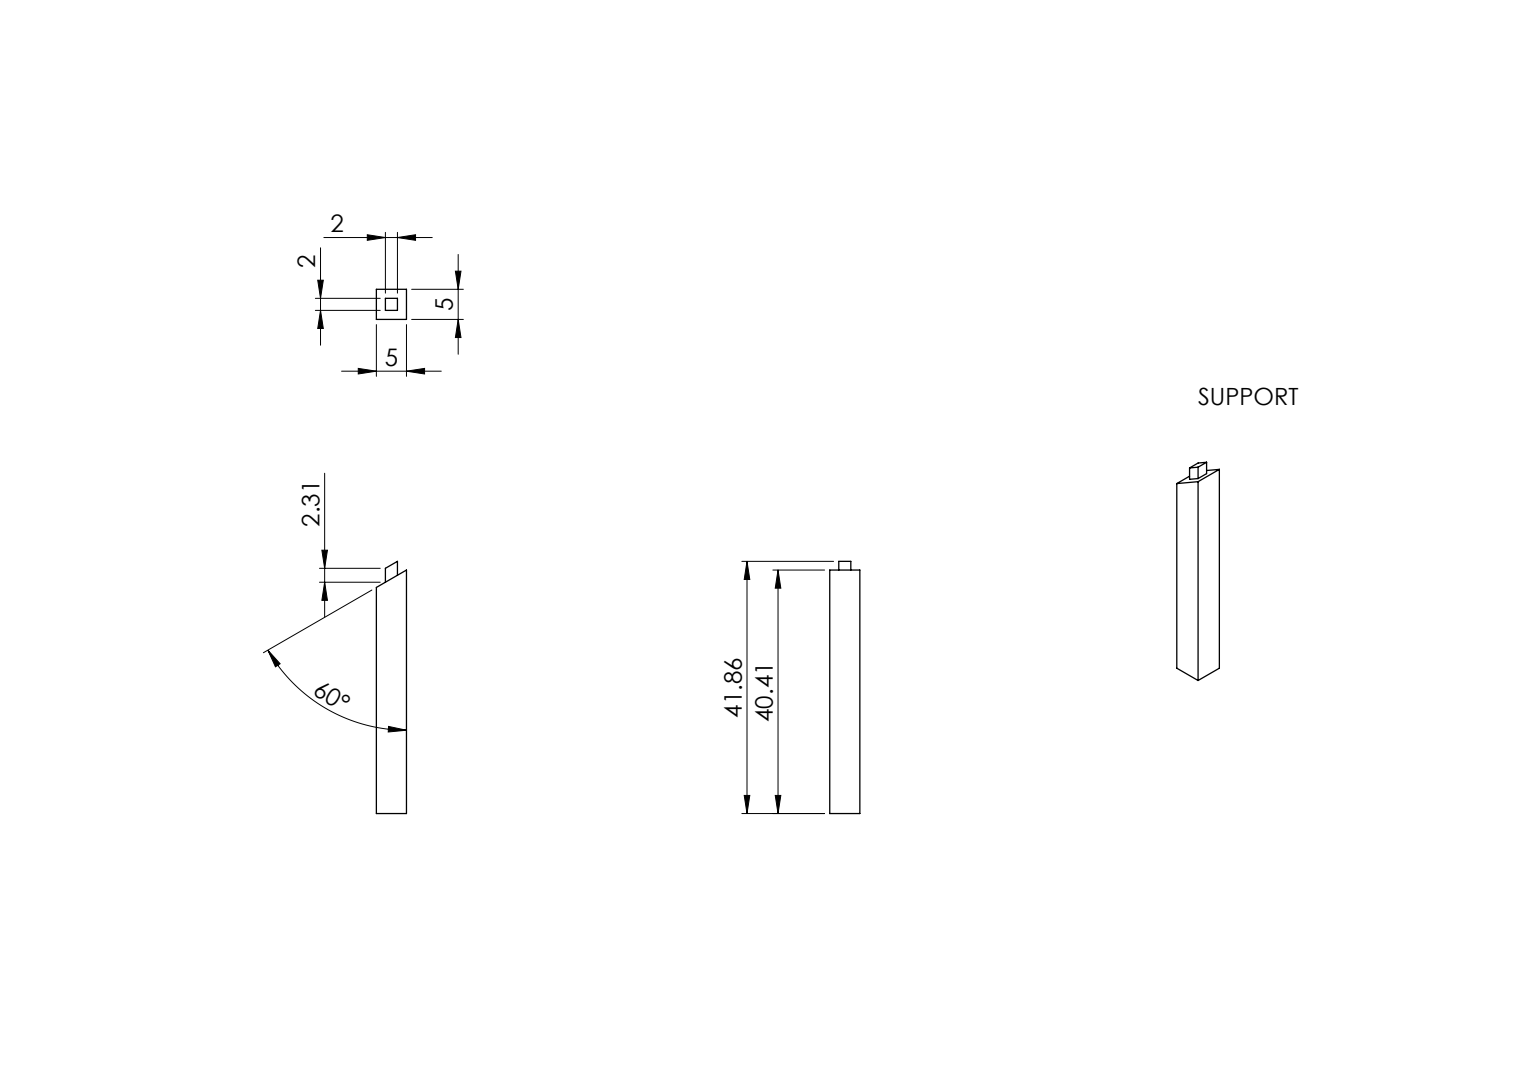
ISO-10303-21;
HEADER;
FILE_DESCRIPTION (('STEP AP214'),
    '1' );
FILE_NAME ('support.step',
    '2026-10-26T05:17:54',
    ( '' ),
    ( '' ),
    'SwSTEP 2.0',
    'SolidWorks 2026',
    '' );
FILE_SCHEMA (( 'AUTOMOTIVE_DESIGN' ));
ENDSEC;

DATA;
#17=CARTESIAN_POINT ( 'NONE',  ( 7.500000000000000000, 34.99999999999999289, -1.499999999999999556 ) ) ;
#43=ORIENTED_EDGE ( 'NONE', *, *, #1360, .T. ) ;
#55=APPLICATION_CONTEXT ( 'automotive_design' ) ;
#65=ORIENTED_EDGE ( 'NONE', *, *, #9345, .T. ) ;
#128=DIRECTION ( 'NONE',  ( 0.000000000000000000, 0.000000000000000000, -1.000000000000000000 ) ) ;
#162=ORIENTED_EDGE ( 'NONE', *, *, #11234, .F. ) ;
#197=DIRECTION ( 'NONE',  ( -0.000000000000000000, -1.000000000000000000, -0.000000000000000000 ) ) ;
#254=EDGE_CURVE ( 'NONE', #5137, #10011, #5741, .T. ) ;
#287=ADVANCED_FACE ( 'NONE', ( #7172 ), #1536, .F. ) ;
#303=DIRECTION ( 'NONE',  ( -1.000000000000000000, 0.000000000000000000, 4.336808689942017243E-16 ) ) ;
#312=ORIENTED_EDGE ( 'NONE', *, *, #4163, .F. ) ;
#338=ADVANCED_FACE ( 'NONE', ( #7108, #5337 ), #2214, .T. ) ;
#342=VECTOR ( 'NONE', #6084, 1000.000000000000000 ) ;
#366=LINE ( 'NONE', #8567, #6016 ) ;
#411=DIRECTION ( 'NONE',  ( -0.000000000000000000, 1.000000000000000000, -0.000000000000000000 ) ) ;
#459=DIRECTION ( 'NONE',  ( 0.000000000000000000, 0.000000000000000000, -1.000000000000000000 ) ) ;
#466=( GEOMETRIC_REPRESENTATION_CONTEXT ( 3 ) GLOBAL_UNCERTAINTY_ASSIGNED_CONTEXT ( ( #584 ) ) GLOBAL_UNIT_ASSIGNED_CONTEXT ( ( #1408, #547, #9650 ) ) REPRESENTATION_CONTEXT ( 'NONE', 'WORKASPACE' ) );
#522=DIRECTION ( 'NONE',  ( -0.000000000000000000, -1.000000000000000000, -0.000000000000000000 ) ) ;
#547=( NAMED_UNIT ( * ) PLANE_ANGLE_UNIT ( ) SI_UNIT ( $, .RADIAN. ) );
#559=DIRECTION ( 'NONE',  ( 1.000000000000000000, -0.000000000000000000, 0.000000000000000000 ) ) ;
#563=ORIENTED_EDGE ( 'NONE', *, *, #5905, .F. ) ;
#584=UNCERTAINTY_MEASURE_WITH_UNIT (LENGTH_MEASURE( 1.000000000000000082E-05 ), #1408, 'distance_accuracy_value', 'NONE');
#592=ORIENTED_EDGE ( 'NONE', *, *, #5905, .T. ) ;
#593=ADVANCED_FACE ( 'NONE', ( #5912, #5791 ), #3774, .T. ) ;
#615=( NAMED_UNIT ( * ) SI_UNIT ( $, .STERADIAN. ) SOLID_ANGLE_UNIT ( ) );
#628=LINE ( 'NONE', #4760, #11001 ) ;
#659=CARTESIAN_POINT ( 'NONE',  ( 6.499999999999999112, 68.39379290111055809, 2.999999999999960032 ) ) ;
#674=DIRECTION ( 'NONE',  ( -0.000000000000000000, 1.000000000000000000, -0.000000000000000000 ) ) ;
#682=CARTESIAN_POINT ( 'NONE',  ( 7.500000000000000000, 30.00000000000000000, 0.000000000000000000 ) ) ;
#692=LINE ( 'NONE', #4702, #11877 ) ;
#733=CARTESIAN_POINT ( 'NONE',  ( -61.00000000000000711, 26.13129029178200469, 0.9999999999999926725 ) ) ;
#790=DIRECTION ( 'NONE',  ( -1.084202172485503571E-16, 0.000000000000000000, 1.000000000000000000 ) ) ;
#872=CYLINDRICAL_SURFACE ( 'NONE', #11788, 1.499999999999999556 ) ;
#904=APPLICATION_CONTEXT ( 'automotive_design' ) ;
#954=ADVANCED_FACE ( 'NONE', ( #9768 ), #6949, .T. ) ;
#969=ORIENTED_EDGE ( 'NONE', *, *, #12016, .T. ) ;
#978=CARTESIAN_POINT ( 'NONE',  ( 9.999999999999994671, 70.41451884327426569, -2.500000000000000000 ) ) ;
#1019=DIRECTION ( 'NONE',  ( 0.000000000000000000, 0.000000000000000000, -1.000000000000000000 ) ) ;
#1027=DIRECTION ( 'NONE',  ( -1.000000000000000000, 0.000000000000000000, 1.084202172485504064E-16 ) ) ;
#1095=EDGE_LOOP ( 'NONE', ( #4761, #6603, #12509, #12056 ) ) ;
#1137=VECTOR ( 'NONE', #8632, 1000.000000000000000 ) ;
#1175=CYLINDRICAL_SURFACE ( 'NONE', #1863, 1.499999999999999556 ) ;
#1187=DIRECTION ( 'NONE',  ( -0.000000000000000000, -1.000000000000000000, -0.000000000000000000 ) ) ;
#1217=CARTESIAN_POINT ( 'NONE',  ( 7.500000000000000000, 34.99999999999999289, 0.000000000000000000 ) ) ;
#1229=DIRECTION ( 'NONE',  ( 0.8660254037844361541, 0.5000000000000042188, 0.000000000000000000 ) ) ;
#1270=CARTESIAN_POINT ( 'NONE',  ( 7.500000000000000000, 34.99999999999999289, 0.000000000000000000 ) ) ;
#1271=EDGE_CURVE ( 'NONE', #8824, #5732, #8757, .T. ) ;
#1360=EDGE_CURVE ( 'NONE', #5732, #10262, #11699, .T. ) ;
#1370=AXIS2_PLACEMENT_3D ( 'NONE', #3051, #11936, #5062 ) ;
#1393=EDGE_CURVE ( 'NONE', #11615, #4578, #5928, .T. ) ;
#1408=( LENGTH_UNIT ( ) NAMED_UNIT ( * ) SI_UNIT ( .MILLI., .METRE. ) );
#1455=CARTESIAN_POINT ( 'NONE',  ( 7.500000000000000000, 34.99999999999999289, 0.000000000000000000 ) ) ;
#1536=CONICAL_SURFACE ( 'NONE', #6345, 1.499999999999999556, 1.029744259999998190 ) ;
#1555=CARTESIAN_POINT ( 'NONE',  ( 6.499999999999999112, 65.10243346208218895, 2.999999999999960920 ) ) ;
#1563=ORIENTED_EDGE ( 'NONE', *, *, #9726, .T. ) ;
#1579=ORIENTED_EDGE ( 'NONE', *, *, #11333, .T. ) ;
#1609=( NAMED_UNIT ( * ) PLANE_ANGLE_UNIT ( ) SI_UNIT ( $, .RADIAN. ) );
#1623=PLANE ( 'NONE',  #1727 ) ;
#1667=DIRECTION ( 'NONE',  ( 0.000000000000000000, 0.000000000000000000, 1.000000000000000000 ) ) ;
#1671=CARTESIAN_POINT ( 'NONE',  ( 8.499999999999998224, 66.25713400046146262, 1.000000000000000444 ) ) ;
#1679=CARTESIAN_POINT ( 'NONE',  ( 5.000000000000005329, 67.52776749732610995, -2.500000000000000000 ) ) ;
#1695=CARTESIAN_POINT ( 'NONE',  ( 9.999999999999994671, 76.58915998087155685, 2.500000000000000444 ) ) ;
#1698=VERTEX_POINT ( 'NONE', #7439 ) ;
#1718=LINE ( 'NONE', #5706, #4125 ) ;
#1727=AXIS2_PLACEMENT_3D ( 'NONE', #9605, #10958, #1815 ) ;
#1732=EDGE_LOOP ( 'NONE', ( #4996, #3921, #6198 ) ) ;
#1765=EDGE_CURVE ( 'NONE', #9740, #3991, #8262, .T. ) ;
#1806=PLANE ( 'NONE',  #1370 ) ;
#1810=VERTEX_POINT ( 'NONE', #1679 ) ;
#1815=DIRECTION ( 'NONE',  ( -0.8660254037844361541, -0.5000000000000042188, 0.000000000000000000 ) ) ;
#1835=ORIENTED_EDGE ( 'NONE', *, *, #11333, .F. ) ;
#1844=ORIENTED_EDGE ( 'NONE', *, *, #11101, .F. ) ;
#1852=AXIS2_PLACEMENT_3D ( 'NONE', #1555, #303, #7378 ) ;
#1863=AXIS2_PLACEMENT_3D ( 'NONE', #4323, #6337, #7327 ) ;
#1908=LINE ( 'NONE', #659, #6411 ) ;
#1928=ADVANCED_FACE ( 'NONE', ( #8928 ), #1806, .F. ) ;
#1951=CLOSED_SHELL ( 'NONE', ( #2139, #6471, #593, #3644, #3730, #1928, #5531, #338, #6814, #6013, #11811, #954, #12893, #7708, #287 ) ) ;
#1963=VECTOR ( 'NONE', #8093, 1000.000000000000114 ) ;
#2028=EDGE_LOOP ( 'NONE', ( #2316, #6397, #9153, #3795 ) ) ;
#2085=AXIS2_PLACEMENT_3D ( 'NONE', #6228, #1187, #128 ) ;
#2139=ADVANCED_FACE ( 'NONE', ( #10235 ), #6382, .F. ) ;
#2214=PLANE ( 'NONE',  #6768 ) ;
#2316=ORIENTED_EDGE ( 'NONE', *, *, #12882, .F. ) ;
#2321=LINE ( 'NONE', #5374, #12344 ) ;
#2327=VECTOR ( 'NONE', #197, 1000.000000000000000 ) ;
#2355=EDGE_LOOP ( 'NONE', ( #6387, #1563, #6766, #2685 ) ) ;
#2399=PRODUCT_DEFINITION_SHAPE ( 'NONE', 'NONE',  #8014 ) ;
#2422=SHAPE_REPRESENTATION ( 'support', ( #5704 ), #466 ) ;
#2446=EDGE_LOOP ( 'NONE', ( #162, #3575, #4707, #65 ) ) ;
#2447=LINE ( 'NONE', #12380, #9210 ) ;
#2545=CARTESIAN_POINT ( 'NONE',  ( 8.500000000000000000, 69.54849343948981755, 2.999999999999918288 ) ) ;
#2610=FACE_OUTER_BOUND ( 'NONE', #7322, .T. ) ;
#2612=DIRECTION ( 'NONE',  ( 0.000000000000000000, 0.000000000000000000, -1.000000000000000000 ) ) ;
#2685=ORIENTED_EDGE ( 'NONE', *, *, #3331, .T. ) ;
#2706=DIRECTION ( 'NONE',  ( 4.336808689942017736E-16, 2.503857664561960972E-16, 1.000000000000000000 ) ) ;
#2799=ORIENTED_EDGE ( 'NONE', *, *, #1271, .T. ) ;
#2818=PLANE ( 'NONE',  #6930 ) ;
#2827=CARTESIAN_POINT ( 'NONE',  ( -62.42520044359213927, 28.59980987105325667, 0.9999999999999924505 ) ) ;
#2828=VERTEX_POINT ( 'NONE', #8029 ) ;
#2894=VECTOR ( 'NONE', #2612, 1000.000000000000000 ) ;
#2903=VECTOR ( 'NONE', #1229, 1000.000000000000114 ) ;
#2917=VECTOR ( 'NONE', #9628, 1000.000000000000000 ) ;
#2995=MECHANICAL_DESIGN_GEOMETRIC_PRESENTATION_REPRESENTATION('',(#9040),#10302);
#3010=EDGE_CURVE ( 'NONE', #7510, #3209, #7171, .T. ) ;
#3014=CARTESIAN_POINT ( 'NONE',  ( 7.500000000000000000, 30.00000000000000000, 1.499999999999999556 ) ) ;
#3027=ORIENTED_EDGE ( 'NONE', *, *, #1765, .F. ) ;
#3051=CARTESIAN_POINT ( 'NONE',  ( 9.999999999999994671, 76.58915998087155685, 2.500000000000000444 ) ) ;
#3052=STYLED_ITEM('',(#12988),#3308);
#3120=ORIENTED_EDGE ( 'NONE', *, *, #4526, .T. ) ;
#3187=ORIENTED_EDGE ( 'NONE', *, *, #10309, .F. ) ;
#3209=VERTEX_POINT ( 'NONE', #5530 ) ;
#3303=ORIENTED_EDGE ( 'NONE', *, *, #1765, .T. ) ;
#3308=MANIFOLD_SOLID_BREP ( 'AdvancedHole1', #1951 ) ;
#3331=EDGE_CURVE ( 'NONE', #11426, #10133, #5874, .T. ) ;
#3353=EDGE_LOOP ( 'NONE', ( #11829, #2799, #43, #6095 ) ) ;
#3391=CARTESIAN_POINT ( 'NONE',  ( -61.00000000000000711, 31.73205080756887142, 0.9999999999999926725 ) ) ;
#3409=SHAPE_DEFINITION_REPRESENTATION ( #2399, #2422 ) ;
#3426=DIRECTION ( 'NONE',  ( -8.673617379884035472E-16, -5.007715329123921945E-16, -1.000000000000000000 ) ) ;
#3480=VECTOR ( 'NONE', #6054, 1000.000000000000114 ) ;
#3555=CARTESIAN_POINT ( 'NONE',  ( 7.500000000000000000, 34.99999999999999289, 0.000000000000000000 ) ) ;
#3559=CIRCLE ( 'NONE', #6250, 1.499999999999999556 ) ;
#3575=ORIENTED_EDGE ( 'NONE', *, *, #9520, .F. ) ;
#3644=ADVANCED_FACE ( 'NONE', ( #5539 ), #6516, .F. ) ;
#3697=EDGE_CURVE ( 'NONE', #10418, #5137, #7506, .T. ) ;
#3714=CARTESIAN_POINT ( 'NONE',  ( 6.499999999999998224, 68.39379290111055809, 0.9999999999999995559 ) ) ;
#3730=ADVANCED_FACE ( 'NONE', ( #8869 ), #11879, .F. ) ;
#3751=DIRECTION ( 'NONE',  ( 1.000000000000000000, 0.000000000000000000, 0.000000000000000000 ) ) ;
#3774=PLANE ( 'NONE',  #9282 ) ;
#3795=ORIENTED_EDGE ( 'NONE', *, *, #4878, .F. ) ;
#3806=DIRECTION ( 'NONE',  ( 1.049727191973304038E-16, -0.5150380737757271898, 0.8571673013836847987 ) ) ;
#3879=ORIENTED_EDGE ( 'NONE', *, *, #4878, .T. ) ;
#3888=VECTOR ( 'NONE', #4836, 1000.000000000000114 ) ;
#3896=ORIENTED_EDGE ( 'NONE', *, *, #1271, .F. ) ;
#3903=FACE_OUTER_BOUND ( 'NONE', #2446, .T. ) ;
#3921=ORIENTED_EDGE ( 'NONE', *, *, #1393, .T. ) ;
#3963=EDGE_CURVE ( 'NONE', #1810, #10261, #9517, .T. ) ;
#3991=VERTEX_POINT ( 'NONE', #8477 ) ;
#4033=CARTESIAN_POINT ( 'NONE',  ( 5.000000000000004441, 76.58915998087155685, 2.500000000000000444 ) ) ;
#4078=VECTOR ( 'NONE', #1019, 1000.000000000000000 ) ;
#4121=EDGE_LOOP ( 'NONE', ( #563, #12287, #11521, #3896 ) ) ;
#4125=VECTOR ( 'NONE', #3751, 1000.000000000000000 ) ;
#4163=EDGE_CURVE ( 'NONE', #1698, #4578, #12048, .T. ) ;
#4212=VERTEX_POINT ( 'NONE', #9823 ) ;
#4289=EDGE_CURVE ( 'NONE', #10418, #11426, #1908, .T. ) ;
#4296=ORIENTED_EDGE ( 'NONE', *, *, #9492, .F. ) ;
#4301=CARTESIAN_POINT ( 'NONE',  ( 8.500000000000000000, 71.85789451624832225, -1.000000000000000666 ) ) ;
#4323=CARTESIAN_POINT ( 'NONE',  ( 7.500000000000000000, 30.00000000000000000, 0.000000000000000000 ) ) ;
#4324=EDGE_CURVE ( 'NONE', #8136, #5732, #1718, .T. ) ;
#4361=EDGE_CURVE ( 'NONE', #1810, #2828, #8027, .T. ) ;
#4378=ORIENTED_EDGE ( 'NONE', *, *, #8402, .T. ) ;
#4379=PRODUCT ( 'support', 'support', '', ( #6596 ) ) ;
#4425=SURFACE_STYLE_USAGE ( .BOTH. , #8673 ) ;
#4490=SURFACE_STYLE_FILL_AREA ( #9588 ) ;
#4501=DIRECTION ( 'NONE',  ( 0.000000000000000000, 0.000000000000000000, -1.000000000000000000 ) ) ;
#4526=EDGE_CURVE ( 'NONE', #11432, #1810, #628, .T. ) ;
#4578=VERTEX_POINT ( 'NONE', #17 ) ;
#4589=CIRCLE ( 'NONE', #2085, 1.499999999999999556 ) ;
#4702=CARTESIAN_POINT ( 'NONE',  ( 5.000000000000004441, 76.58915998087155685, 2.500000000000000444 ) ) ;
#4707=ORIENTED_EDGE ( 'NONE', *, *, #11101, .T. ) ;
#4711=ORIENTED_EDGE ( 'NONE', *, *, #3331, .F. ) ;
#4734=PLANE ( 'NONE',  #7090 ) ;
#4739=AXIS2_PLACEMENT_3D ( 'NONE', #4033, #5795, #11938 ) ;
#4760=CARTESIAN_POINT ( 'NONE',  ( 8.923698042205888470, 69.79311561821251075, -2.500000000000000000 ) ) ;
#4761=ORIENTED_EDGE ( 'NONE', *, *, #3963, .F. ) ;
#4810=ORIENTED_EDGE ( 'NONE', *, *, #3697, .T. ) ;
#4824=DIRECTION ( 'NONE',  ( 0.000000000000000000, 0.000000000000000000, 1.000000000000000000 ) ) ;
#4836=DIRECTION ( 'NONE',  ( 0.8660254037844361541, 0.5000000000000042188, -9.389466242107214363E-17 ) ) ;
#4878=EDGE_CURVE ( 'NONE', #4212, #10011, #9586, .T. ) ;
#4886=DIRECTION ( 'NONE',  ( 1.000000000000000000, 0.000000000000000000, 0.000000000000000000 ) ) ;
#4898=EDGE_LOOP ( 'NONE', ( #10984, #3879, #10531, #5569 ) ) ;
#4901=FACE_OUTER_BOUND ( 'NONE', #6011, .T. ) ;
#4958=VECTOR ( 'NONE', #411, 1000.000000000000000 ) ;
#4996=ORIENTED_EDGE ( 'NONE', *, *, #8402, .F. ) ;
#5062=DIRECTION ( 'NONE',  ( 0.000000000000000000, 0.000000000000000000, 1.000000000000000000 ) ) ;
#5132=MECHANICAL_DESIGN_GEOMETRIC_PRESENTATION_REPRESENTATION('',(#3052),#6173);
#5137=VERTEX_POINT ( 'NONE', #7092 ) ;
#5147=EDGE_LOOP ( 'NONE', ( #7533, #4378, #9977 ) ) ;
#5262=DIRECTION ( 'NONE',  ( -0.000000000000000000, -1.000000000000000000, -0.000000000000000000 ) ) ;
#5285=DIRECTION ( 'NONE',  ( -1.000000000000000000, -0.000000000000000000, -0.000000000000000000 ) ) ;
#5316=LINE ( 'NONE', #12187, #2327 ) ;
#5337=FACE_OUTER_BOUND ( 'NONE', #9194, .T. ) ;
#5360=EDGE_LOOP ( 'NONE', ( #312, #6700, #3303, #1844 ) ) ;
#5374=CARTESIAN_POINT ( 'NONE',  ( 7.500000000000000000, 30.00000000000000000, -1.499999999999999556 ) ) ;
#5442=DIRECTION ( 'NONE',  ( -0.000000000000000000, -1.000000000000000000, -0.000000000000000000 ) ) ;
#5452=VECTOR ( 'NONE', #2706, 1000.000000000000000 ) ;
#5465=DIRECTION ( 'NONE',  ( -0.000000000000000000, -1.000000000000000000, -0.000000000000000000 ) ) ;
#5467=ORIENTED_EDGE ( 'NONE', *, *, #4289, .F. ) ;
#5475=LINE ( 'NONE', #2545, #7580 ) ;
#5530=CARTESIAN_POINT ( 'NONE',  ( 6.499999999999997335, 70.70319397786906279, -1.000000000000000888 ) ) ;
#5531=ADVANCED_FACE ( 'NONE', ( #12305 ), #12370, .F. ) ;
#5539=FACE_OUTER_BOUND ( 'NONE', #1095, .T. ) ;
#5563=CARTESIAN_POINT ( 'NONE',  ( 5.000000000000004441, 76.58915998087155685, -2.500000000000000000 ) ) ;
#5569=ORIENTED_EDGE ( 'NONE', *, *, #3697, .F. ) ;
#5596=FILL_AREA_STYLE_COLOUR ( '', #8642 ) ;
#5603=CARTESIAN_POINT ( 'NONE',  ( 5.000000000000005329, 67.52776749732610995, 2.500000000000000444 ) ) ;
#5627=ORIENTED_EDGE ( 'NONE', *, *, #8035, .T. ) ;
#5665=DIRECTION ( 'NONE',  ( 0.000000000000000000, 0.000000000000000000, -1.000000000000000000 ) ) ;
#5679=PRODUCT_DEFINITION_CONTEXT ( 'detailed design', #904, 'design' ) ;
#5704=AXIS2_PLACEMENT_3D ( 'NONE', #8997, #4824, #4886 ) ;
#5706=CARTESIAN_POINT ( 'NONE',  ( 5.000000000000004441, 30.00000000000000000, 2.500000000000000444 ) ) ;
#5732=VERTEX_POINT ( 'NONE', #8826 ) ;
#5734=ORIENTED_EDGE ( 'NONE', *, *, #7188, .T. ) ;
#5741=LINE ( 'NONE', #3391, #1963 ) ;
#5791=FACE_BOUND ( 'NONE', #2355, .T. ) ;
#5795=DIRECTION ( 'NONE',  ( 0.000000000000000000, 0.000000000000000000, -1.000000000000000000 ) ) ;
#5874=LINE ( 'NONE', #5999, #3888 ) ;
#5905=EDGE_CURVE ( 'NONE', #10261, #8824, #6071, .T. ) ;
#5912=FACE_OUTER_BOUND ( 'NONE', #5918, .T. ) ;
#5918=EDGE_LOOP ( 'NONE', ( #3120, #12904, #592, #5734 ) ) ;
#5928=LINE ( 'NONE', #10842, #10757 ) ;
#5975=EDGE_CURVE ( 'NONE', #10262, #2828, #366, .T. ) ;
#5979=VECTOR ( 'NONE', #1667, 1000.000000000000000 ) ;
#5999=CARTESIAN_POINT ( 'NONE',  ( -62.42520044359213927, 28.59980987105325667, -0.9999999999999928946 ) ) ;
#6011=EDGE_LOOP ( 'NONE', ( #4711, #969, #10869, #3187 ) ) ;
#6013=ADVANCED_FACE ( 'NONE', ( #10456 ), #8431, .T. ) ;
#6016=VECTOR ( 'NONE', #5285, 1000.000000000000000 ) ;
#6054=DIRECTION ( 'NONE',  ( -0.8660254037844361541, -0.5000000000000042188, 9.389466242107213130E-17 ) ) ;
#6071=LINE ( 'NONE', #8953, #2903 ) ;
#6076=EDGE_LOOP ( 'NONE', ( #10405, #5627, #6929, #10969 ) ) ;
#6084=DIRECTION ( 'NONE',  ( -0.000000000000000000, -1.000000000000000000, -0.000000000000000000 ) ) ;
#6095=ORIENTED_EDGE ( 'NONE', *, *, #8035, .F. ) ;
#6114=EDGE_CURVE ( 'NONE', #10261, #8136, #692, .T. ) ;
#6161=VECTOR ( 'NONE', #3806, 1000.000000000000227 ) ;
#6173=( GEOMETRIC_REPRESENTATION_CONTEXT ( 3 ) GLOBAL_UNCERTAINTY_ASSIGNED_CONTEXT ( ( #12082 ) ) GLOBAL_UNIT_ASSIGNED_CONTEXT ( ( #7526, #9616, #6663 ) ) REPRESENTATION_CONTEXT ( 'NONE', 'WORKASPACE' ) );
#6198=ORIENTED_EDGE ( 'NONE', *, *, #9520, .T. ) ;
#6200=LINE ( 'NONE', #7621, #10695 ) ;
#6228=CARTESIAN_POINT ( 'NONE',  ( 7.500000000000000000, 30.00000000000000000, 0.000000000000000000 ) ) ;
#6250=AXIS2_PLACEMENT_3D ( 'NONE', #3555, #522, #9366 ) ;
#6337=DIRECTION ( 'NONE',  ( -0.000000000000000000, -1.000000000000000000, -0.000000000000000000 ) ) ;
#6345=AXIS2_PLACEMENT_3D ( 'NONE', #1217, #10247, #9199 ) ;
#6382=CONICAL_SURFACE ( 'NONE', #11401, 1.499999999999999556, 1.029744259999998190 ) ;
#6387=ORIENTED_EDGE ( 'NONE', *, *, #12882, .T. ) ;
#6397=ORIENTED_EDGE ( 'NONE', *, *, #10309, .T. ) ;
#6410=DIRECTION ( 'NONE',  ( 1.000000000000000000, 0.000000000000000000, -0.000000000000000000 ) ) ;
#6411=VECTOR ( 'NONE', #9760, 1000.000000000000000 ) ;
#6471=ADVANCED_FACE ( 'NONE', ( #8315 ), #1175, .F. ) ;
#6495=CARTESIAN_POINT ( 'NONE',  ( 9.999999999999994671, 76.58915998087155685, -2.500000000000000000 ) ) ;
#6516=PLANE ( 'NONE',  #11824 ) ;
#6523=DIRECTION ( 'NONE',  ( 8.673617379884034486E-16, 5.007715329123921945E-16, 1.000000000000000000 ) ) ;
#6596=PRODUCT_CONTEXT ( 'NONE', #55, 'mechanical' ) ;
#6603=ORIENTED_EDGE ( 'NONE', *, *, #4361, .T. ) ;
#6623=DIRECTION ( 'NONE',  ( -0.000000000000000000, -1.000000000000000000, -0.000000000000000000 ) ) ;
#6636=AXIS2_PLACEMENT_3D ( 'NONE', #5563, #9558, #6410 ) ;
#6637=SHAPE_REPRESENTATION_RELATIONSHIP ( 'NONE' , 'NONE' ,  #2422, #7935 ) ;
#6654=CARTESIAN_POINT ( 'NONE',  ( 9.999999999999994671, 70.41451884327426569, 2.500000000000000444 ) ) ;
#6663=( NAMED_UNIT ( * ) SI_UNIT ( $, .STERADIAN. ) SOLID_ANGLE_UNIT ( ) );
#6700=ORIENTED_EDGE ( 'NONE', *, *, #11234, .T. ) ;
#6766=ORIENTED_EDGE ( 'NONE', *, *, #4289, .T. ) ;
#6768=AXIS2_PLACEMENT_3D ( 'NONE', #11091, #9332, #12214 ) ;
#6814=ADVANCED_FACE ( 'NONE', ( #12522 ), #4734, .T. ) ;
#6916=DIRECTION ( 'NONE',  ( 0.000000000000000000, -0.5150380737757271898, -0.8571673013836847987 ) ) ;
#6929=ORIENTED_EDGE ( 'NONE', *, *, #5975, .T. ) ;
#6930=AXIS2_PLACEMENT_3D ( 'NONE', #9997, #8947, #1027 ) ;
#6949=PLANE ( 'NONE',  #9499 ) ;
#7008=CARTESIAN_POINT ( 'NONE',  ( 5.000000000000004441, 76.58915998087155685, -2.500000000000000000 ) ) ;
#7031=AXIS2_PLACEMENT_3D ( 'NONE', #1455, #5442, #459 ) ;
#7090=AXIS2_PLACEMENT_3D ( 'NONE', #733, #790, #7676 ) ;
#7092=CARTESIAN_POINT ( 'NONE',  ( 6.499999999999998224, 70.70319397786906279, 1.000000000000000000 ) ) ;
#7108=FACE_BOUND ( 'NONE', #10385, .T. ) ;
#7171=LINE ( 'NONE', #10179, #3480 ) ;
#7172=FACE_OUTER_BOUND ( 'NONE', #1732, .T. ) ;
#7188=EDGE_CURVE ( 'NONE', #8824, #11432, #11631, .T. ) ;
#7279=ORIENTED_EDGE ( 'NONE', *, *, #11152, .T. ) ;
#7322=EDGE_LOOP ( 'NONE', ( #7813, #7279, #11627, #1579 ) ) ;
#7327=DIRECTION ( 'NONE',  ( 0.000000000000000000, 0.000000000000000000, -1.000000000000000000 ) ) ;
#7378=DIRECTION ( 'NONE',  ( 4.336808689942017243E-16, 0.000000000000000000, 1.000000000000000000 ) ) ;
#7431=( LENGTH_UNIT ( ) NAMED_UNIT ( * ) SI_UNIT ( .MILLI., .METRE. ) );
#7439=CARTESIAN_POINT ( 'NONE',  ( 7.500000000000000000, 34.99999999999999289, 1.499999999999999556 ) ) ;
#7476=CARTESIAN_POINT ( 'NONE',  ( 6.499999999999999112, 68.39379290111055809, -1.000000000000000222 ) ) ;
#7506=LINE ( 'NONE', #8992, #12249 ) ;
#7510=VERTEX_POINT ( 'NONE', #4301 ) ;
#7525=ORIENTED_EDGE ( 'NONE', *, *, #1360, .F. ) ;
#7526=( LENGTH_UNIT ( ) NAMED_UNIT ( * ) SI_UNIT ( .MILLI., .METRE. ) );
#7533=ORIENTED_EDGE ( 'NONE', *, *, #1393, .F. ) ;
#7577=DIRECTION ( 'NONE',  ( -0.000000000000000000, -1.000000000000000000, -0.000000000000000000 ) ) ;
#7580=VECTOR ( 'NONE', #6523, 1000.000000000000000 ) ;
#7609=PRODUCT_DEFINITION_FORMATION_WITH_SPECIFIED_SOURCE ( 'ANY', '', #4379, .NOT_KNOWN. ) ;
#7618=CARTESIAN_POINT ( 'NONE',  ( 5.000000000000004441, 67.52776749732610995, 2.500000000000000444 ) ) ;
#7621=CARTESIAN_POINT ( 'NONE',  ( 6.499999999999997335, 65.10243346208218895, -1.000000000000000888 ) ) ;
#7625=VECTOR ( 'NONE', #6623, 1000.000000000000000 ) ;
#7676=DIRECTION ( 'NONE',  ( 1.000000000000000000, 0.000000000000000000, 1.084202172485503571E-16 ) ) ;
#7708=ADVANCED_FACE ( 'NONE', ( #3903 ), #872, .F. ) ;
#7759=DIRECTION ( 'NONE',  ( -0.000000000000000000, 1.000000000000000000, -0.000000000000000000 ) ) ;
#7779=ORIENTED_EDGE ( 'NONE', *, *, #4324, .F. ) ;
#7802=DIRECTION ( 'NONE',  ( 1.000000000000000000, 0.000000000000000000, -8.673617379884034486E-16 ) ) ;
#7813=ORIENTED_EDGE ( 'NONE', *, *, #254, .T. ) ;
#7935=ADVANCED_BREP_SHAPE_REPRESENTATION ( '', ( #3308, #5704 ), #466 ) ;
#7952=DIRECTION ( 'NONE',  ( -0.5000000000000043299, 0.8660254037844362651, 0.000000000000000000 ) ) ;
#7959=DIRECTION ( 'NONE',  ( -0.8660254037844361541, -0.5000000000000042188, 0.000000000000000000 ) ) ;
#8014=PRODUCT_DEFINITION ( 'UNKNOWN', '', #7609, #5679 ) ;
#8027=LINE ( 'NONE', #7008, #342 ) ;
#8029=CARTESIAN_POINT ( 'NONE',  ( 5.000000000000004441, 30.00000000000000000, -2.500000000000000000 ) ) ;
#8035=EDGE_CURVE ( 'NONE', #11432, #10262, #8538, .T. ) ;
#8049=ORIENTED_EDGE ( 'NONE', *, *, #9345, .F. ) ;
#8093=DIRECTION ( 'NONE',  ( 0.8660254037844361541, 0.5000000000000042188, 9.389466242107209433E-17 ) ) ;
#8097=CARTESIAN_POINT ( 'NONE',  ( 8.500000000000000000, 69.54849343948981755, -1.000000000000000666 ) ) ;
#8136=VERTEX_POINT ( 'NONE', #11982 ) ;
#8227=CARTESIAN_POINT ( 'NONE',  ( 8.499999999999998224, 71.85789451624832225, 1.000000000000000444 ) ) ;
#8262=CIRCLE ( 'NONE', #12653, 1.499999999999999556 ) ;
#8315=FACE_OUTER_BOUND ( 'NONE', #5360, .T. ) ;
#8402=EDGE_CURVE ( 'NONE', #11615, #1698, #10727, .T. ) ;
#8431=PLANE ( 'NONE',  #1852 ) ;
#8477=CARTESIAN_POINT ( 'NONE',  ( 7.500000000000000000, 30.00000000000000000, -1.499999999999999556 ) ) ;
#8538=LINE ( 'NONE', #6495, #7625 ) ;
#8567=CARTESIAN_POINT ( 'NONE',  ( 5.000000000000004441, 30.00000000000000000, -2.500000000000000000 ) ) ;
#8583=UNCERTAINTY_MEASURE_WITH_UNIT (LENGTH_MEASURE( 1.000000000000000082E-05 ), #7431, 'distance_accuracy_value', 'NONE');
#8618=LINE ( 'NONE', #12797, #12133 ) ;
#8630=CARTESIAN_POINT ( 'NONE',  ( 9.999999999999994671, 70.41451884327426569, 2.500000000000000444 ) ) ;
#8632=DIRECTION ( 'NONE',  ( -0.000000000000000000, -1.000000000000000000, -0.000000000000000000 ) ) ;
#8642=COLOUR_RGB ( '',0.8941176470588234615, 0.8941176470588234615, 0.8941176470588234615 ) ;
#8673=SURFACE_SIDE_STYLE ('',( #4490 ) ) ;
#8736=CARTESIAN_POINT ( 'NONE',  ( -60.00000000000000000, 30.00000000000000000, 3.000000000000000000 ) ) ;
#8757=LINE ( 'NONE', #1695, #1137 ) ;
#8824=VERTEX_POINT ( 'NONE', #8630 ) ;
#8826=CARTESIAN_POINT ( 'NONE',  ( 9.999999999999994671, 30.00000000000000000, 2.500000000000000444 ) ) ;
#8869=FACE_OUTER_BOUND ( 'NONE', #4121, .T. ) ;
#8928=FACE_OUTER_BOUND ( 'NONE', #3353, .T. ) ;
#8947=DIRECTION ( 'NONE',  ( -1.084202172485504064E-16, 0.000000000000000000, -1.000000000000000000 ) ) ;
#8953=CARTESIAN_POINT ( 'NONE',  ( 8.923698042205888470, 69.79311561821251075, 2.500000000000000444 ) ) ;
#8959=LINE ( 'NONE', #2827, #12110 ) ;
#8992=CARTESIAN_POINT ( 'NONE',  ( 6.499999999999998224, 65.10243346208218895, 1.000000000000000000 ) ) ;
#8997=CARTESIAN_POINT ( 'NONE',  ( 0.000000000000000000, 0.000000000000000000, 0.000000000000000000 ) ) ;
#9040=STYLED_ITEM ( 'NONE', ( #10573 ), #7935 ) ;
#9092=ORIENTED_EDGE ( 'NONE', *, *, #5975, .F. ) ;
#9127=EDGE_LOOP ( 'NONE', ( #5467, #4810, #1835, #12054 ) ) ;
#9153=ORIENTED_EDGE ( 'NONE', *, *, #11152, .F. ) ;
#9194=EDGE_LOOP ( 'NONE', ( #4296, #9092, #7525, #7779 ) ) ;
#9199=DIRECTION ( 'NONE',  ( 0.000000000000000000, 0.000000000000000000, -1.000000000000000000 ) ) ;
#9210=VECTOR ( 'NONE', #3426, 1000.000000000000000 ) ;
#9251=DIRECTION ( 'NONE',  ( 0.000000000000000000, 0.000000000000000000, -1.000000000000000000 ) ) ;
#9282=AXIS2_PLACEMENT_3D ( 'NONE', #8736, #7952, #9781 ) ;
#9332=DIRECTION ( 'NONE',  ( 0.000000000000000000, -1.000000000000000000, 0.000000000000000000 ) ) ;
#9345=EDGE_CURVE ( 'NONE', #3991, #9740, #4589, .T. ) ;
#9366=DIRECTION ( 'NONE',  ( 0.000000000000000000, 0.000000000000000000, -1.000000000000000000 ) ) ;
#9492=EDGE_CURVE ( 'NONE', #2828, #8136, #10611, .T. ) ;
#9499=AXIS2_PLACEMENT_3D ( 'NONE', #10812, #7802, #12658 ) ;
#9517=LINE ( 'NONE', #7618, #5979 ) ;
#9520=EDGE_CURVE ( 'NONE', #4578, #1698, #3559, .T. ) ;
#9536=CARTESIAN_POINT ( 'NONE',  ( 5.000000000000004441, 76.58915998087155685, 2.500000000000000444 ) ) ;
#9558=DIRECTION ( 'NONE',  ( 0.000000000000000000, 0.000000000000000000, 1.000000000000000000 ) ) ;
#9586=LINE ( 'NONE', #1671, #4958 ) ;
#9588=FILL_AREA_STYLE ('',( #5596 ) ) ;
#9605=CARTESIAN_POINT ( 'NONE',  ( -28.99038105676692112, 50.21281292110204930, 0.000000000000000000 ) ) ;
#9616=( NAMED_UNIT ( * ) PLANE_ANGLE_UNIT ( ) SI_UNIT ( $, .RADIAN. ) );
#9628=DIRECTION ( 'NONE',  ( -0.000000000000000000, -0.000000000000000000, 1.000000000000000000 ) ) ;
#9650=( NAMED_UNIT ( * ) SI_UNIT ( $, .STERADIAN. ) SOLID_ANGLE_UNIT ( ) );
#9726=EDGE_CURVE ( 'NONE', #4212, #10418, #8959, .T. ) ;
#9740=VERTEX_POINT ( 'NONE', #3014 ) ;
#9759=CARTESIAN_POINT ( 'NONE',  ( 6.499999999999999112, 70.70319397786906279, 2.999999999999960920 ) ) ;
#9760=DIRECTION ( 'NONE',  ( -4.336808689942017243E-16, -2.503857664561960972E-16, -1.000000000000000000 ) ) ;
#9768=FACE_OUTER_BOUND ( 'NONE', #2028, .T. ) ;
#9781=DIRECTION ( 'NONE',  ( -0.8660254037844361541, -0.5000000000000042188, 0.000000000000000000 ) ) ;
#9823=CARTESIAN_POINT ( 'NONE',  ( 8.499999999999998224, 69.54849343948981755, 1.000000000000000000 ) ) ;
#9977=ORIENTED_EDGE ( 'NONE', *, *, #4163, .T. ) ;
#9997=CARTESIAN_POINT ( 'NONE',  ( -61.00000000000000711, 26.13129029178200469, -0.9999999999999931166 ) ) ;
#10011=VERTEX_POINT ( 'NONE', #8227 ) ;
#10133=VERTEX_POINT ( 'NONE', #8097 ) ;
#10140=CARTESIAN_POINT ( 'NONE',  ( 7.500000000000000000, 35.90129092583966752, 0.000000000000000000 ) ) ;
#10179=CARTESIAN_POINT ( 'NONE',  ( -61.00000000000000711, 31.73205080756887142, -0.9999999999999931166 ) ) ;
#10235=FACE_OUTER_BOUND ( 'NONE', #5147, .T. ) ;
#10247=DIRECTION ( 'NONE',  ( -0.000000000000000000, -1.000000000000000000, -0.000000000000000000 ) ) ;
#10261=VERTEX_POINT ( 'NONE', #5603 ) ;
#10262=VERTEX_POINT ( 'NONE', #10699 ) ;
#10302=( GEOMETRIC_REPRESENTATION_CONTEXT ( 3 ) GLOBAL_UNCERTAINTY_ASSIGNED_CONTEXT ( ( #8583 ) ) GLOBAL_UNIT_ASSIGNED_CONTEXT ( ( #7431, #1609, #615 ) ) REPRESENTATION_CONTEXT ( 'NONE', 'WORKASPACE' ) );
#10309=EDGE_CURVE ( 'NONE', #10133, #7510, #8618, .T. ) ;
#10356=DIRECTION ( 'NONE',  ( -0.000000000000000000, -1.000000000000000000, -0.000000000000000000 ) ) ;
#10385=EDGE_LOOP ( 'NONE', ( #8049, #3027 ) ) ;
#10405=ORIENTED_EDGE ( 'NONE', *, *, #4526, .F. ) ;
#10415=CARTESIAN_POINT ( 'NONE',  ( 5.000000000000004441, 30.00000000000000000, 2.500000000000000444 ) ) ;
#10418=VERTEX_POINT ( 'NONE', #3714 ) ;
#10456=FACE_OUTER_BOUND ( 'NONE', #9127, .T. ) ;
#10531=ORIENTED_EDGE ( 'NONE', *, *, #254, .F. ) ;
#10534=DIRECTION ( 'NONE',  ( -0.8660254037844361541, -0.5000000000000042188, -9.389466242107209433E-17 ) ) ;
#10573=PRESENTATION_STYLE_ASSIGNMENT (( #4425 ) ) ;
#10611=LINE ( 'NONE', #10415, #2917 ) ;
#10695=VECTOR ( 'NONE', #674, 1000.000000000000000 ) ;
#10699=CARTESIAN_POINT ( 'NONE',  ( 9.999999999999994671, 30.00000000000000000, -2.500000000000000000 ) ) ;
#10727=LINE ( 'NONE', #10916, #6161 ) ;
#10757=VECTOR ( 'NONE', #6916, 1000.000000000000227 ) ;
#10812=CARTESIAN_POINT ( 'NONE',  ( 8.500000000000000000, 66.25713400046146262, 2.999999999999919620 ) ) ;
#10842=CARTESIAN_POINT ( 'NONE',  ( 7.500000000000000000, 34.99999999999999289, -1.499999999999999556 ) ) ;
#10869=ORIENTED_EDGE ( 'NONE', *, *, #3010, .F. ) ;
#10916=CARTESIAN_POINT ( 'NONE',  ( 7.500000000000000000, 34.99999999999999289, 1.499999999999999556 ) ) ;
#10958=DIRECTION ( 'NONE',  ( -0.5000000000000043299, 0.8660254037844362651, 0.000000000000000000 ) ) ;
#10969=ORIENTED_EDGE ( 'NONE', *, *, #4361, .F. ) ;
#10984=ORIENTED_EDGE ( 'NONE', *, *, #9726, .F. ) ;
#11001=VECTOR ( 'NONE', #7959, 1000.000000000000114 ) ;
#11011=CARTESIAN_POINT ( 'NONE',  ( 7.500000000000000000, 30.00000000000000000, 0.000000000000000000 ) ) ;
#11091=CARTESIAN_POINT ( 'NONE',  ( 0.000000000000000000, 30.00000000000000000, 0.000000000000000000 ) ) ;
#11101=EDGE_CURVE ( 'NONE', #4578, #3991, #2321, .T. ) ;
#11152=EDGE_CURVE ( 'NONE', #10011, #7510, #2447, .T. ) ;
#11234=EDGE_CURVE ( 'NONE', #1698, #9740, #5316, .T. ) ;
#11333=EDGE_CURVE ( 'NONE', #3209, #5137, #11527, .T. ) ;
#11401=AXIS2_PLACEMENT_3D ( 'NONE', #1270, #5262, #9251 ) ;
#11426=VERTEX_POINT ( 'NONE', #7476 ) ;
#11432=VERTEX_POINT ( 'NONE', #978 ) ;
#11521=ORIENTED_EDGE ( 'NONE', *, *, #4324, .T. ) ;
#11527=LINE ( 'NONE', #9759, #5452 ) ;
#11572=CARTESIAN_POINT ( 'NONE',  ( 9.999999999999994671, 30.00000000000000000, 2.500000000000000444 ) ) ;
#11615=VERTEX_POINT ( 'NONE', #10140 ) ;
#11627=ORIENTED_EDGE ( 'NONE', *, *, #3010, .T. ) ;
#11631=LINE ( 'NONE', #6654, #2894 ) ;
#11699=LINE ( 'NONE', #11572, #4078 ) ;
#11788=AXIS2_PLACEMENT_3D ( 'NONE', #11011, #11810, #11873 ) ;
#11810=DIRECTION ( 'NONE',  ( -0.000000000000000000, -1.000000000000000000, -0.000000000000000000 ) ) ;
#11811=ADVANCED_FACE ( 'NONE', ( #4901 ), #2818, .T. ) ;
#11824=AXIS2_PLACEMENT_3D ( 'NONE', #9536, #559, #4501 ) ;
#11829=ORIENTED_EDGE ( 'NONE', *, *, #7188, .F. ) ;
#11873=DIRECTION ( 'NONE',  ( 0.000000000000000000, 0.000000000000000000, -1.000000000000000000 ) ) ;
#11877=VECTOR ( 'NONE', #7577, 1000.000000000000000 ) ;
#11879=PLANE ( 'NONE',  #4739 ) ;
#11936=DIRECTION ( 'NONE',  ( -1.000000000000000000, 0.000000000000000000, 0.000000000000000000 ) ) ;
#11938=DIRECTION ( 'NONE',  ( -1.000000000000000000, 0.000000000000000000, -0.000000000000000000 ) ) ;
#11982=CARTESIAN_POINT ( 'NONE',  ( 5.000000000000004441, 30.00000000000000000, 2.500000000000000444 ) ) ;
#12016=EDGE_CURVE ( 'NONE', #11426, #3209, #6200, .T. ) ;
#12048=CIRCLE ( 'NONE', #7031, 1.499999999999999556 ) ;
#12054=ORIENTED_EDGE ( 'NONE', *, *, #12016, .F. ) ;
#12056=ORIENTED_EDGE ( 'NONE', *, *, #6114, .F. ) ;
#12082=UNCERTAINTY_MEASURE_WITH_UNIT (LENGTH_MEASURE( 1.000000000000000082E-05 ), #7526, 'distance_accuracy_value', 'NONE');
#12110=VECTOR ( 'NONE', #10534, 1000.000000000000114 ) ;
#12133=VECTOR ( 'NONE', #7759, 1000.000000000000000 ) ;
#12187=CARTESIAN_POINT ( 'NONE',  ( 7.500000000000000000, 30.00000000000000000, 1.499999999999999556 ) ) ;
#12214=DIRECTION ( 'NONE',  ( 0.000000000000000000, -0.000000000000000000, -1.000000000000000000 ) ) ;
#12249=VECTOR ( 'NONE', #12798, 1000.000000000000000 ) ;
#12287=ORIENTED_EDGE ( 'NONE', *, *, #6114, .T. ) ;
#12305=FACE_OUTER_BOUND ( 'NONE', #6076, .T. ) ;
#12344=VECTOR ( 'NONE', #10356, 1000.000000000000000 ) ;
#12370=PLANE ( 'NONE',  #6636 ) ;
#12380=CARTESIAN_POINT ( 'NONE',  ( 8.500000000000000000, 71.85789451624832225, 2.999999999999919620 ) ) ;
#12509=ORIENTED_EDGE ( 'NONE', *, *, #9492, .T. ) ;
#12522=FACE_OUTER_BOUND ( 'NONE', #4898, .T. ) ;
#12653=AXIS2_PLACEMENT_3D ( 'NONE', #682, #5465, #5665 ) ;
#12658=DIRECTION ( 'NONE',  ( -8.673617379884034486E-16, 0.000000000000000000, -1.000000000000000000 ) ) ;
#12797=CARTESIAN_POINT ( 'NONE',  ( 8.500000000000000000, 66.25713400046146262, -1.000000000000000666 ) ) ;
#12798=DIRECTION ( 'NONE',  ( -0.000000000000000000, 1.000000000000000000, -0.000000000000000000 ) ) ;
#12882=EDGE_CURVE ( 'NONE', #10133, #4212, #5475, .T. ) ;
#12893=ADVANCED_FACE ( 'NONE', ( #2610 ), #1623, .T. ) ;
#12904=ORIENTED_EDGE ( 'NONE', *, *, #3963, .T. ) ;
#12982=COLOUR_RGB('Light Blue',0.38,0.62,0.78);
#12983=FILL_AREA_STYLE_COLOUR('',#12982);
#12984=FILL_AREA_STYLE('',(#12983));
#12985=SURFACE_STYLE_FILL_AREA(#12984);
#12986=SURFACE_SIDE_STYLE('',(#12985));
#12987=SURFACE_STYLE_USAGE(.BOTH.,#12986);
#12988=PRESENTATION_STYLE_ASSIGNMENT((#12987));
ENDSEC;
END-ISO-10303-21;
